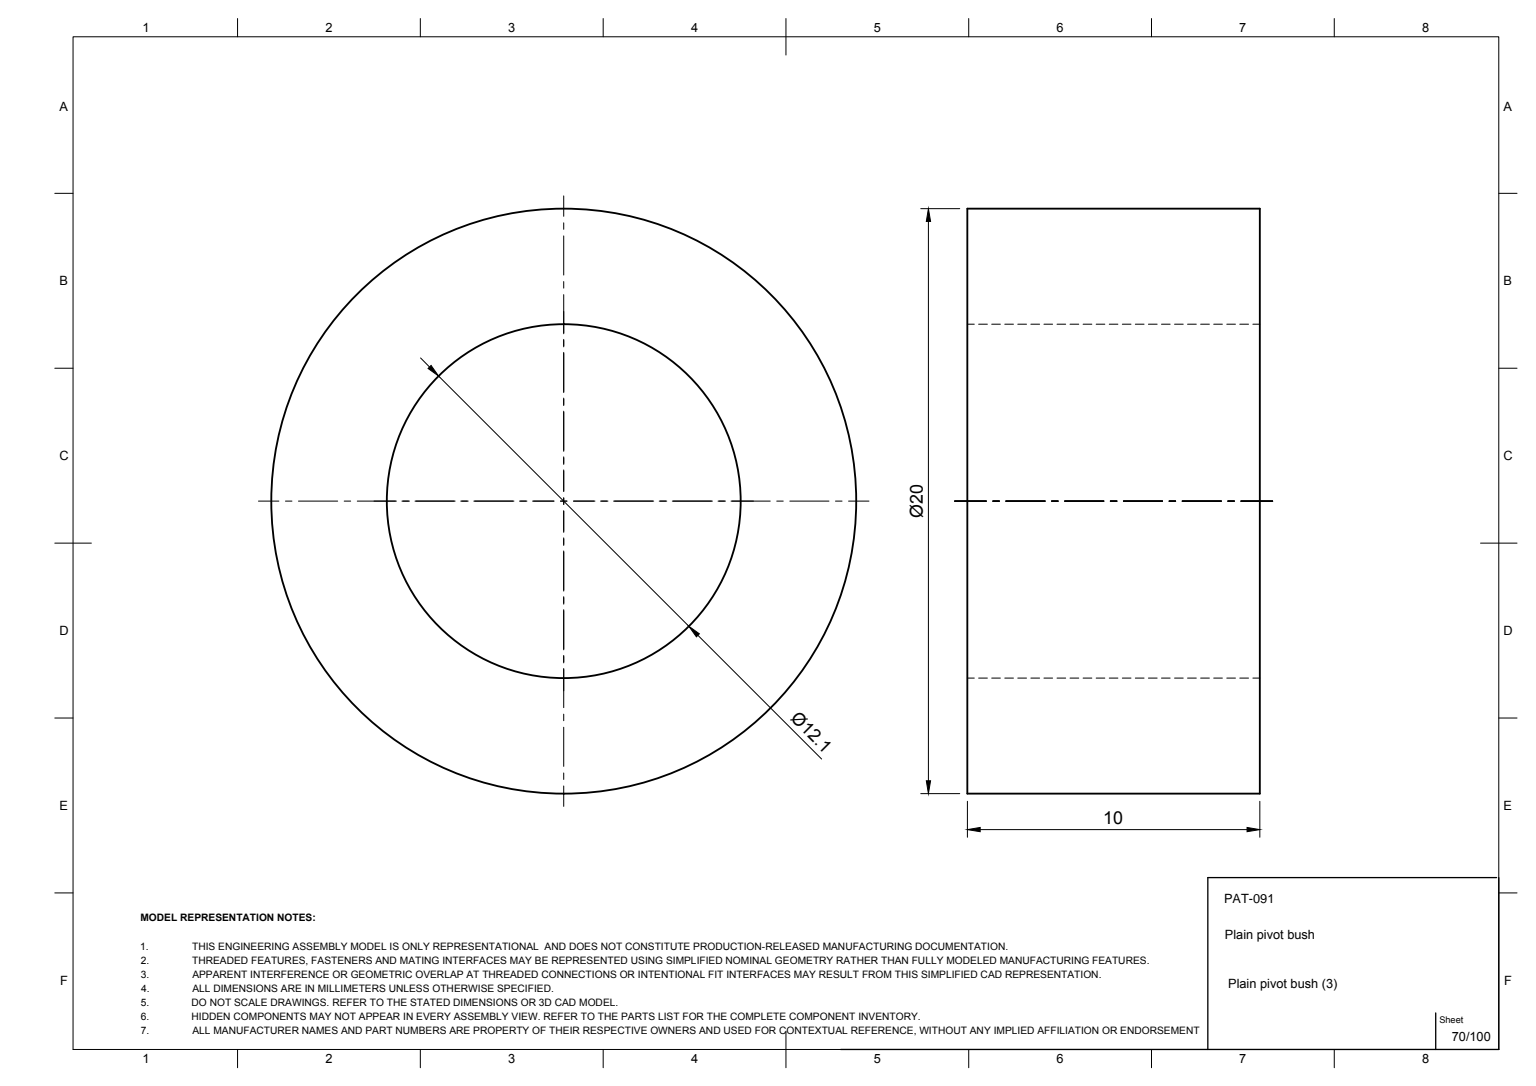
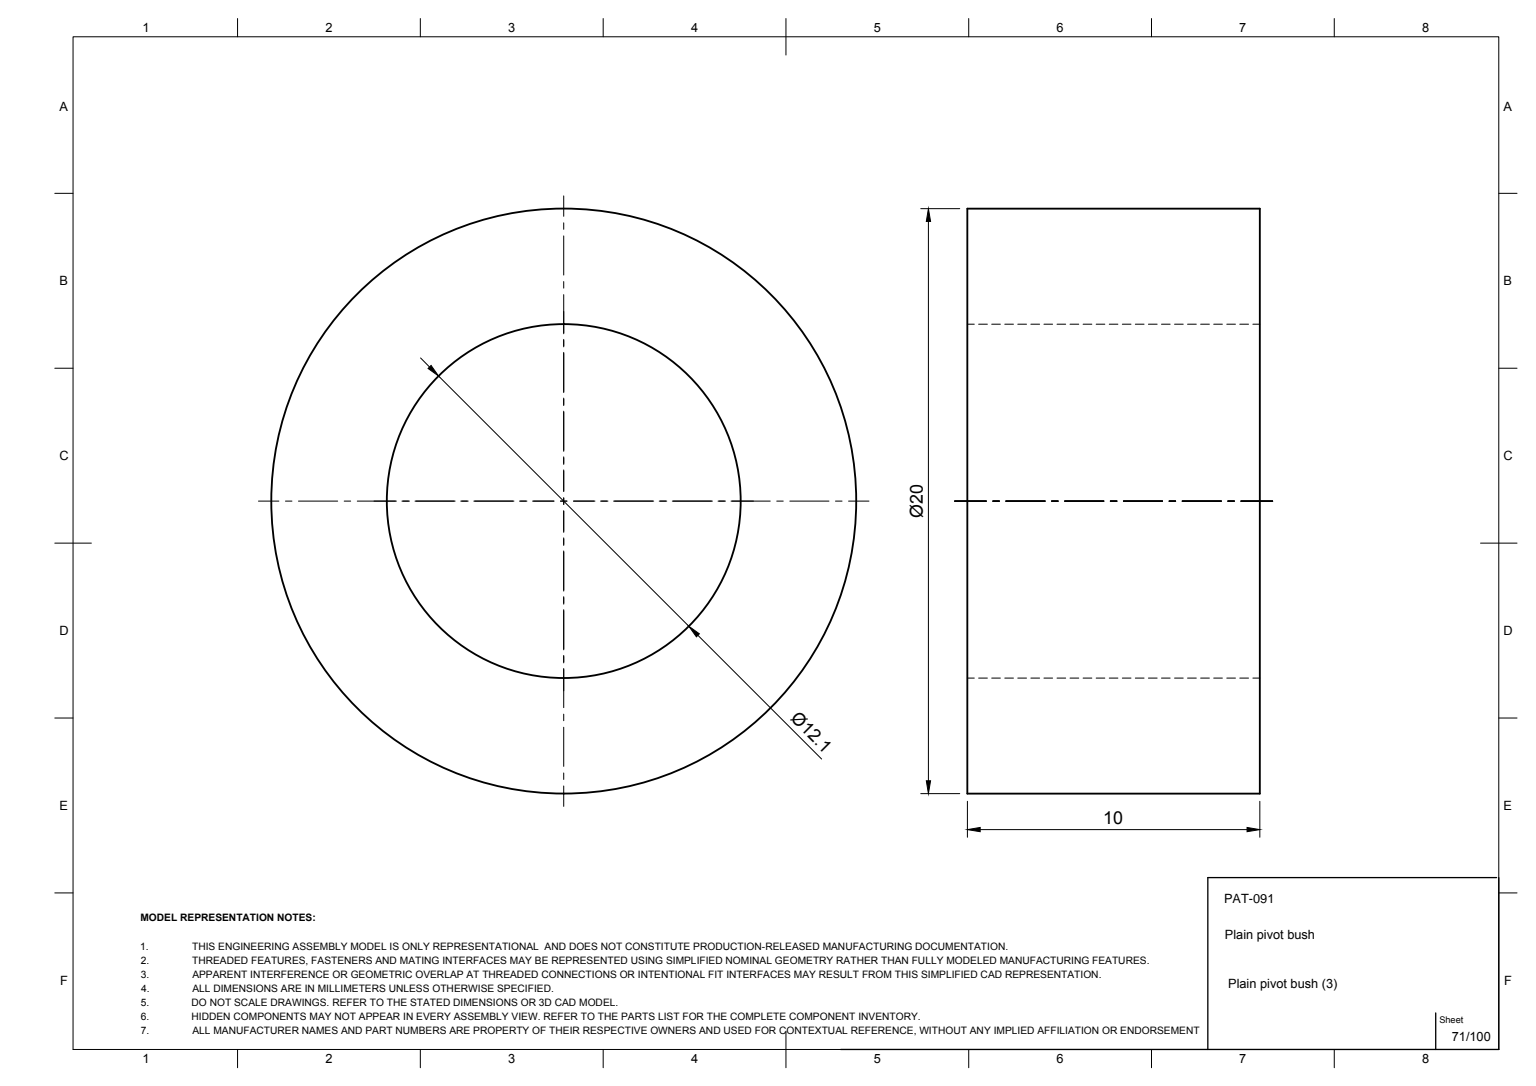
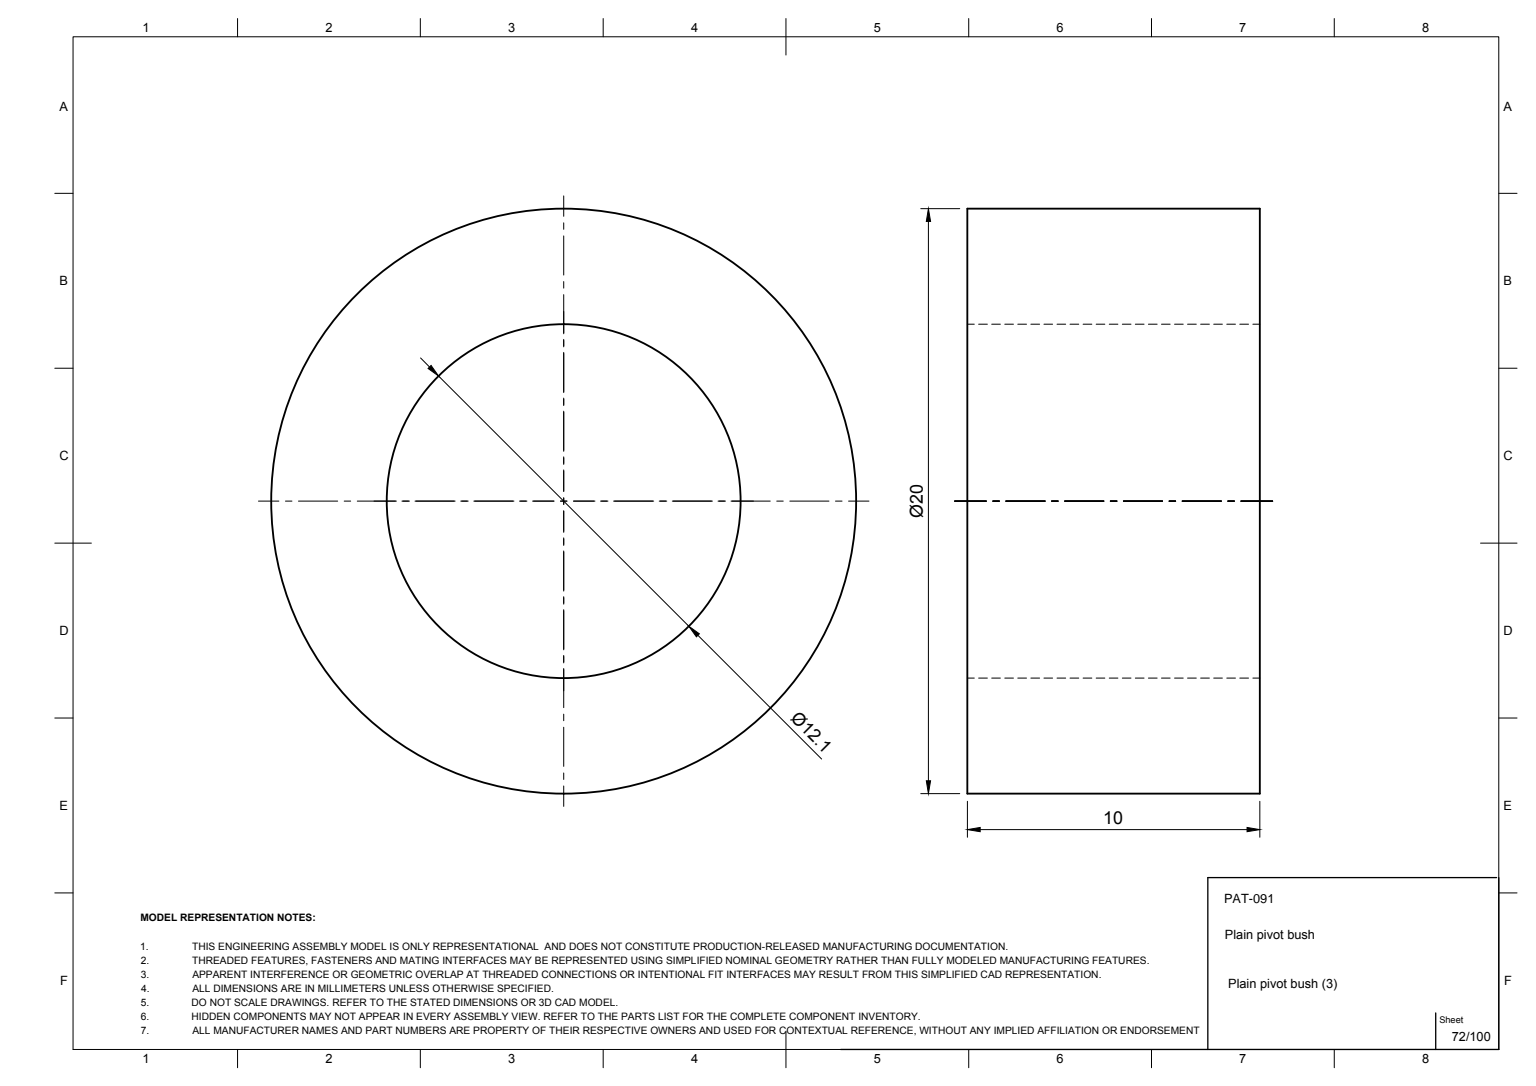
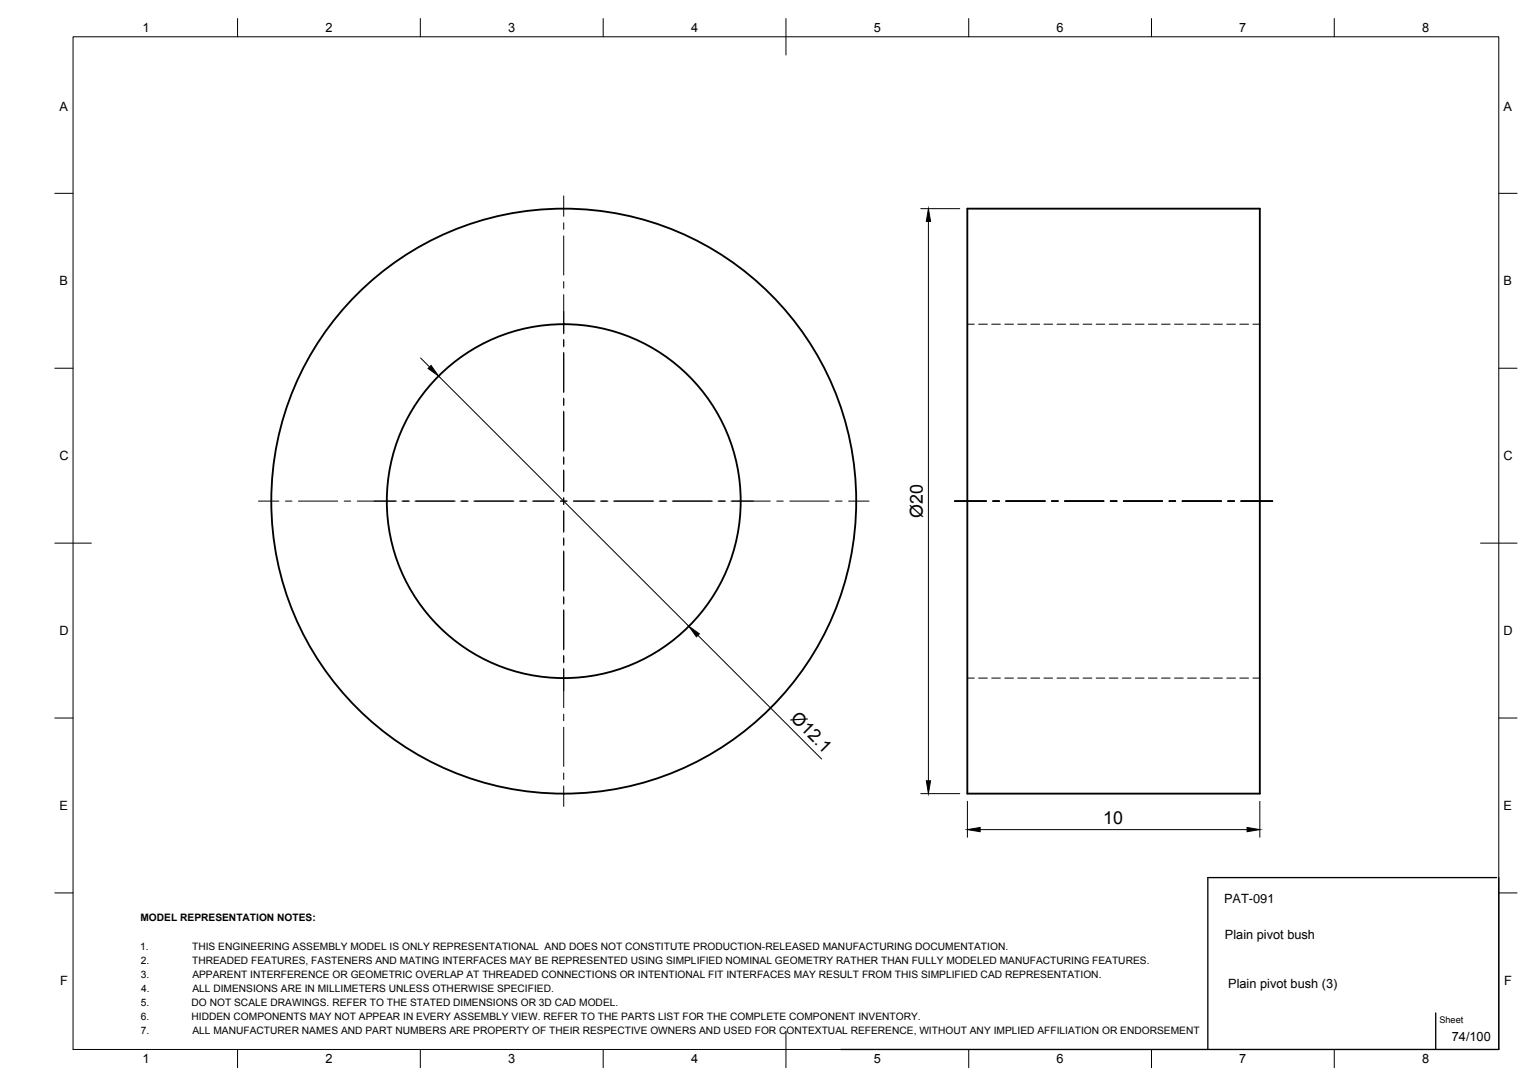
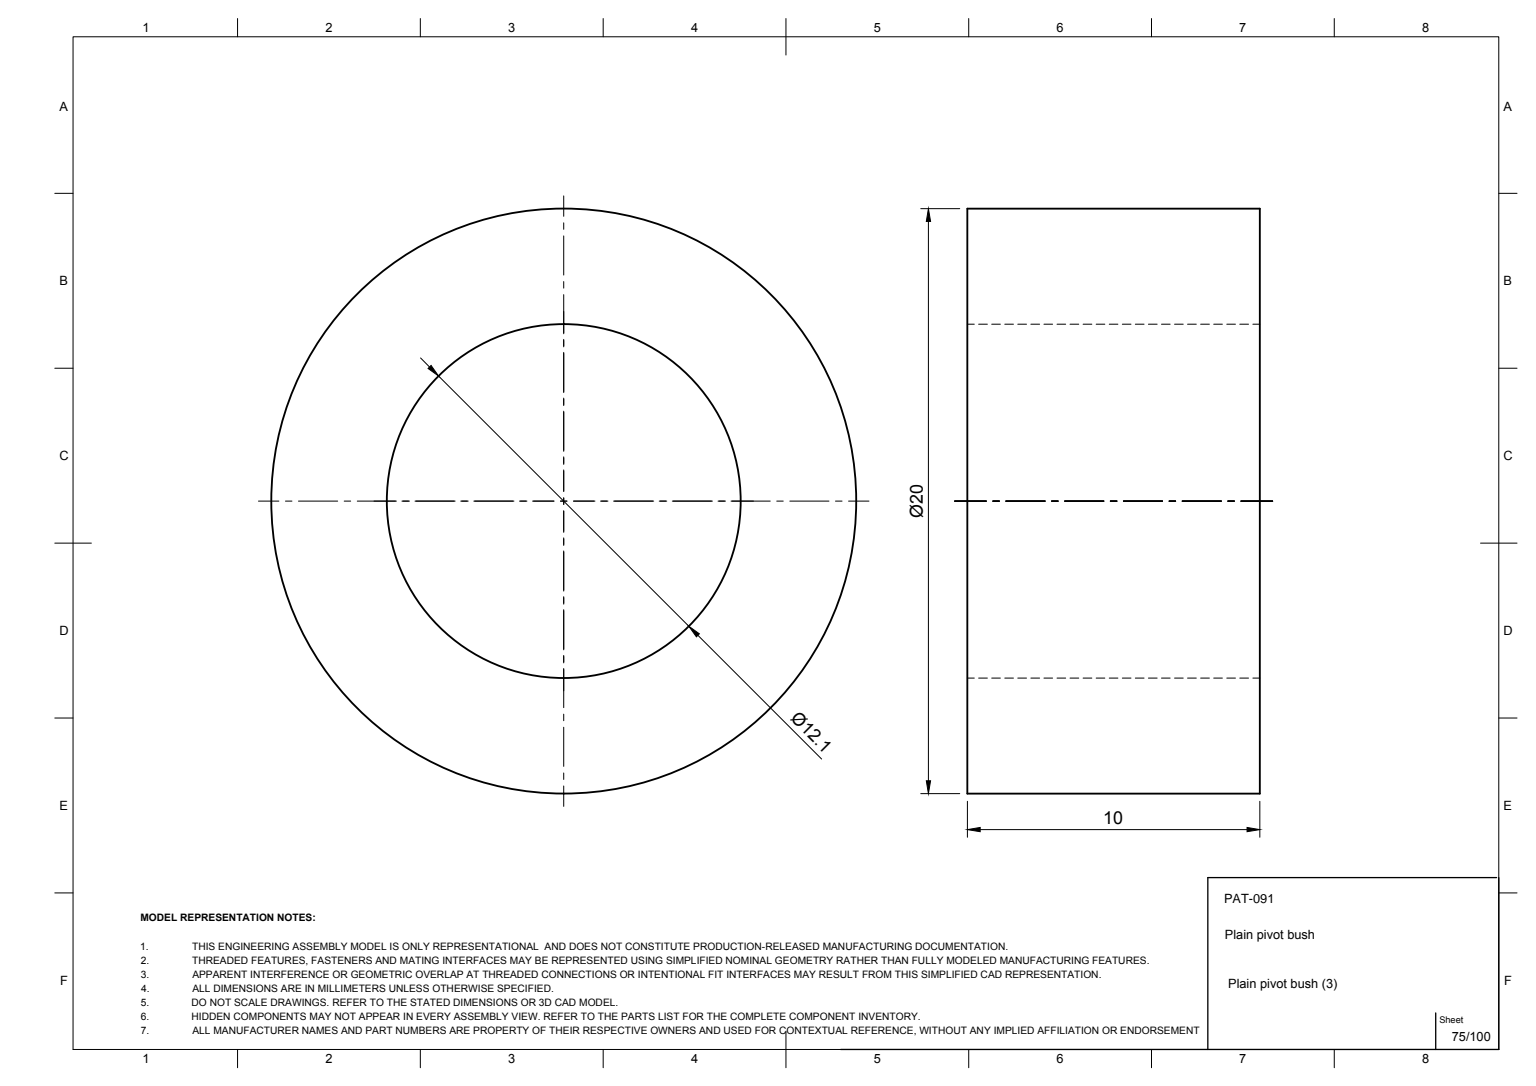
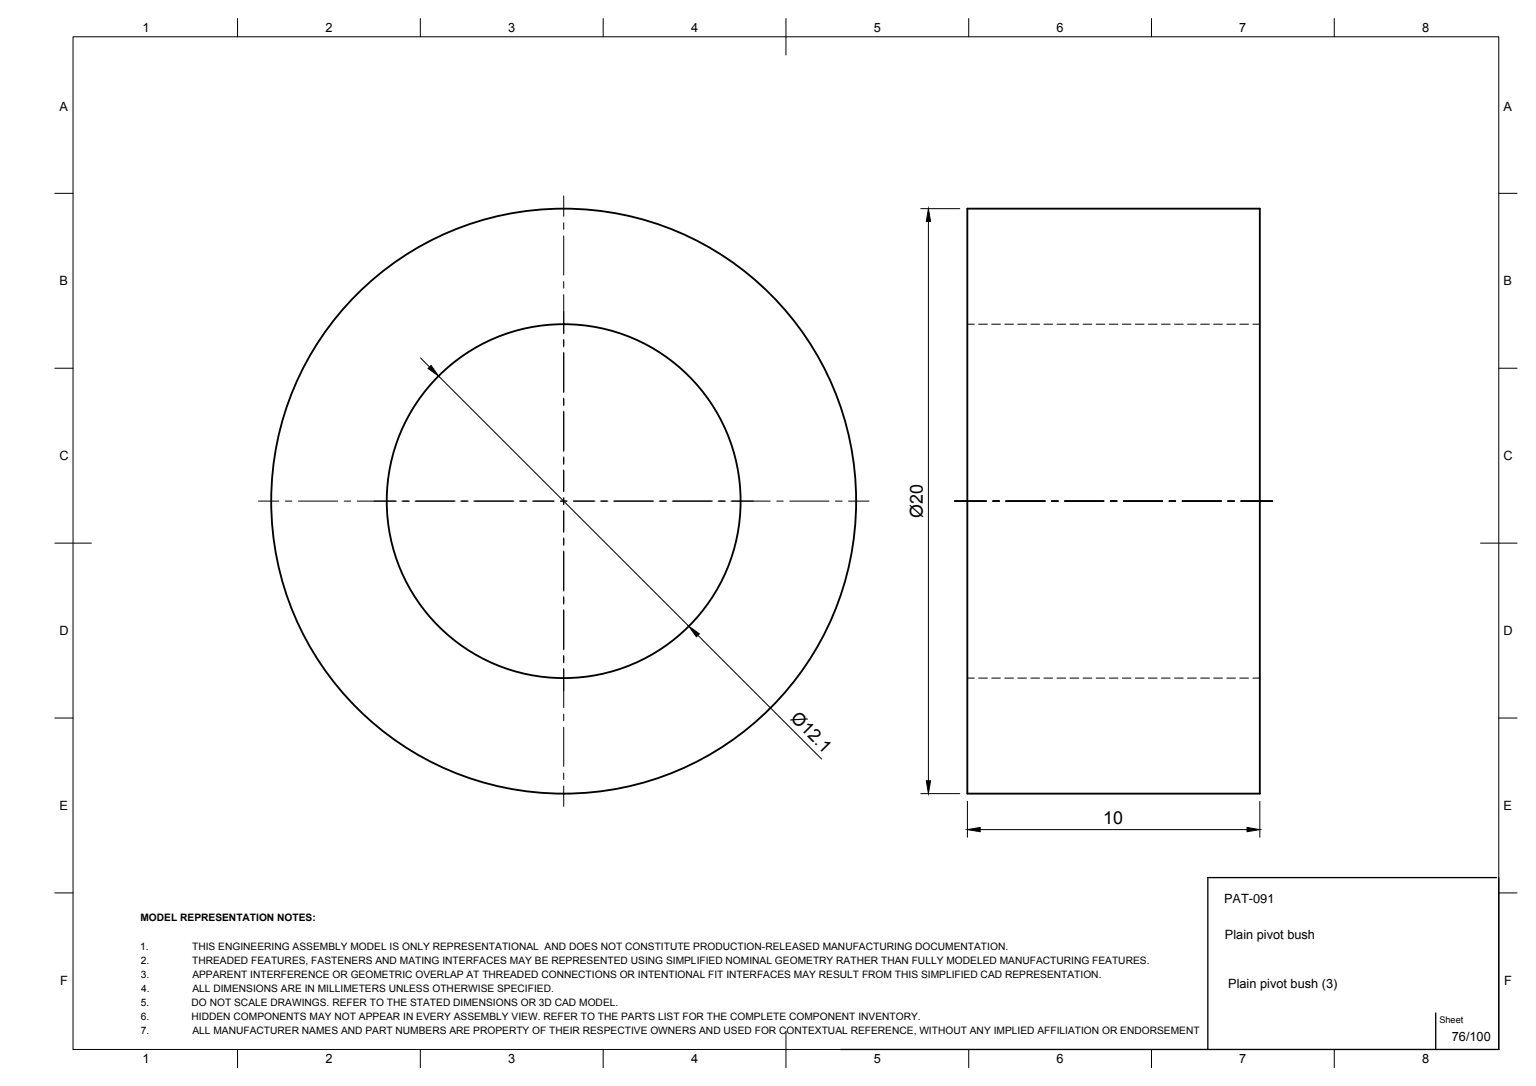
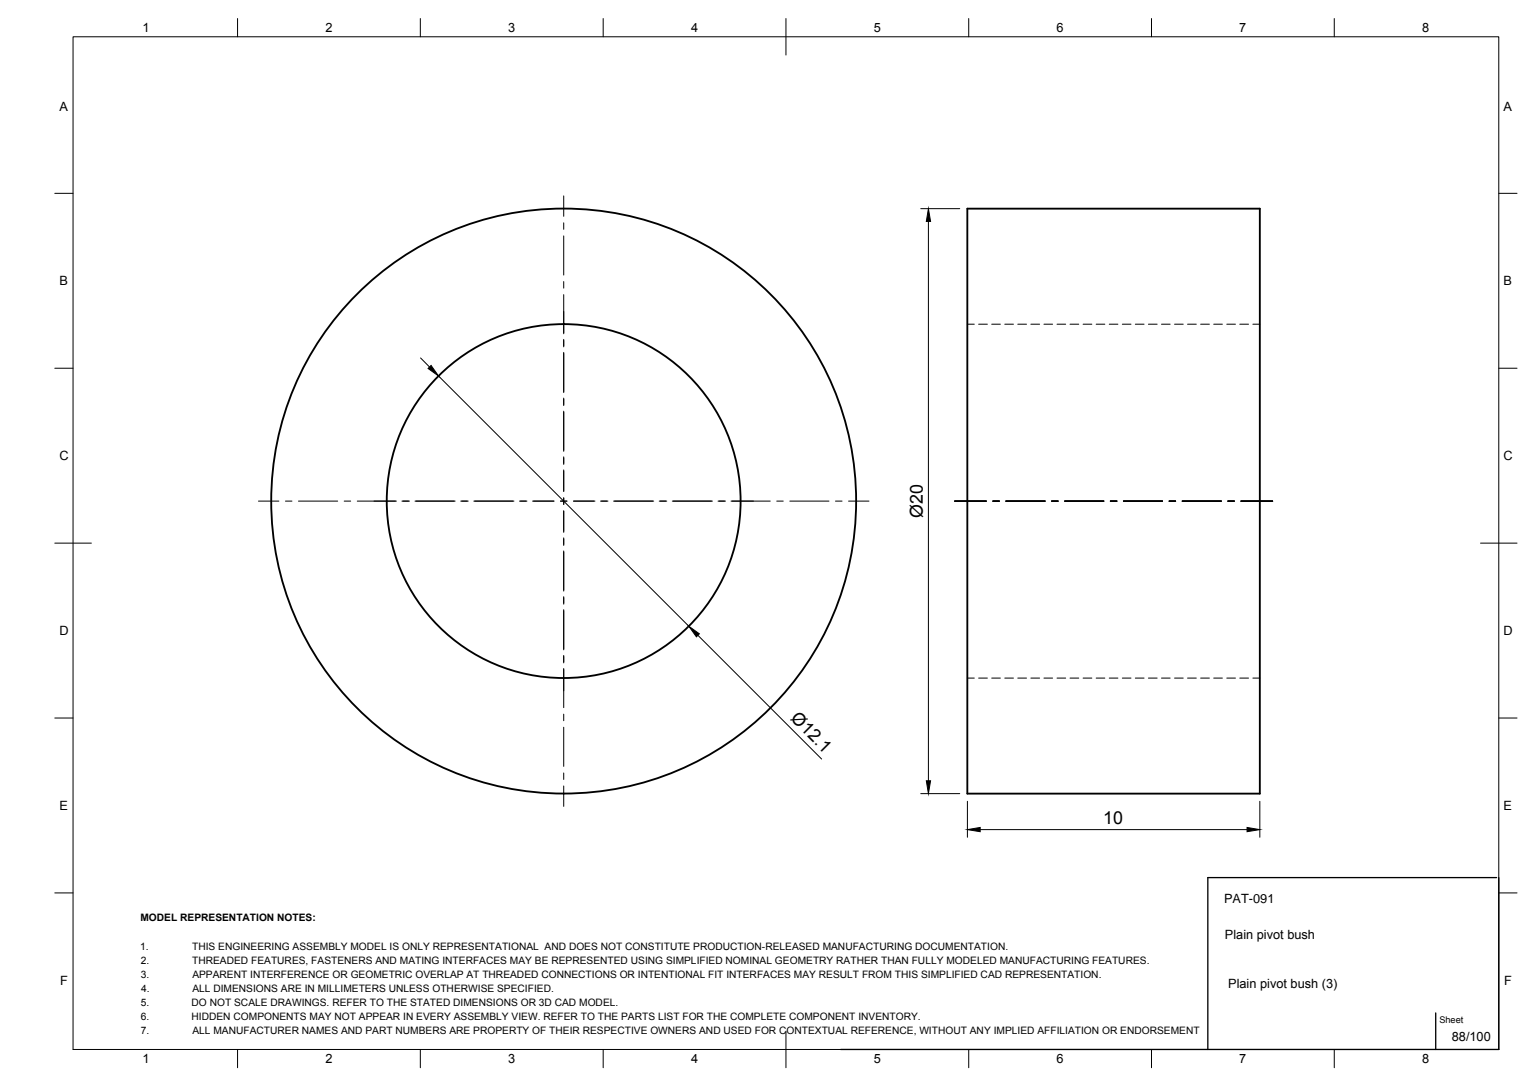
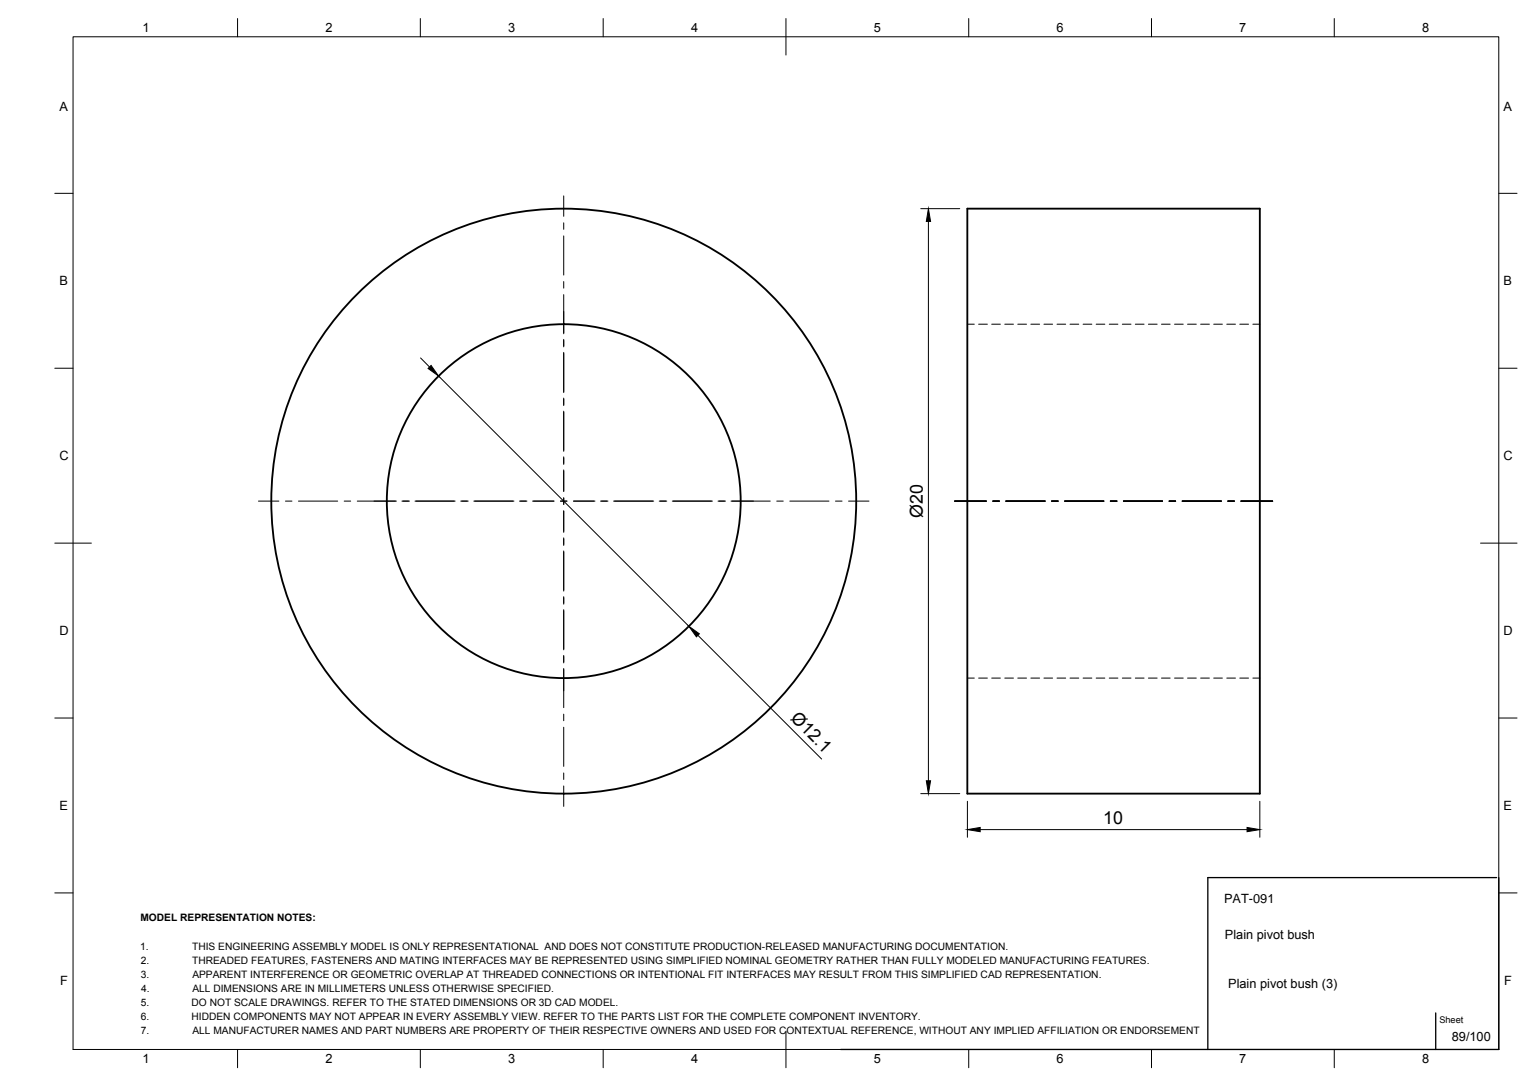
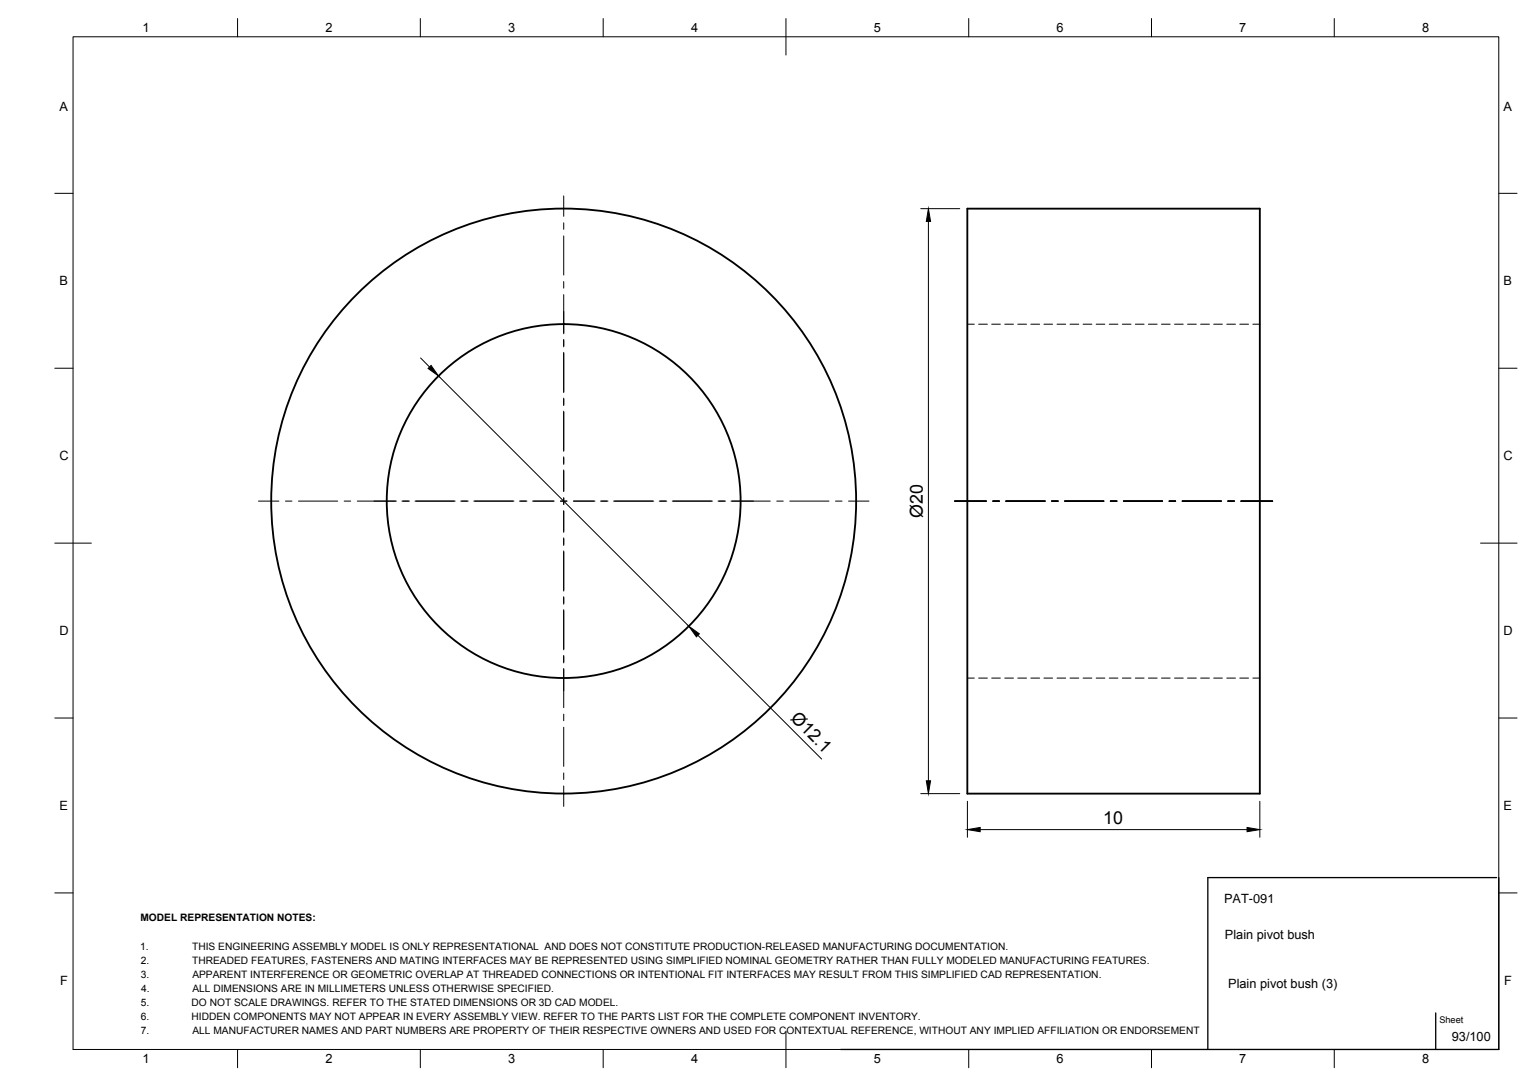
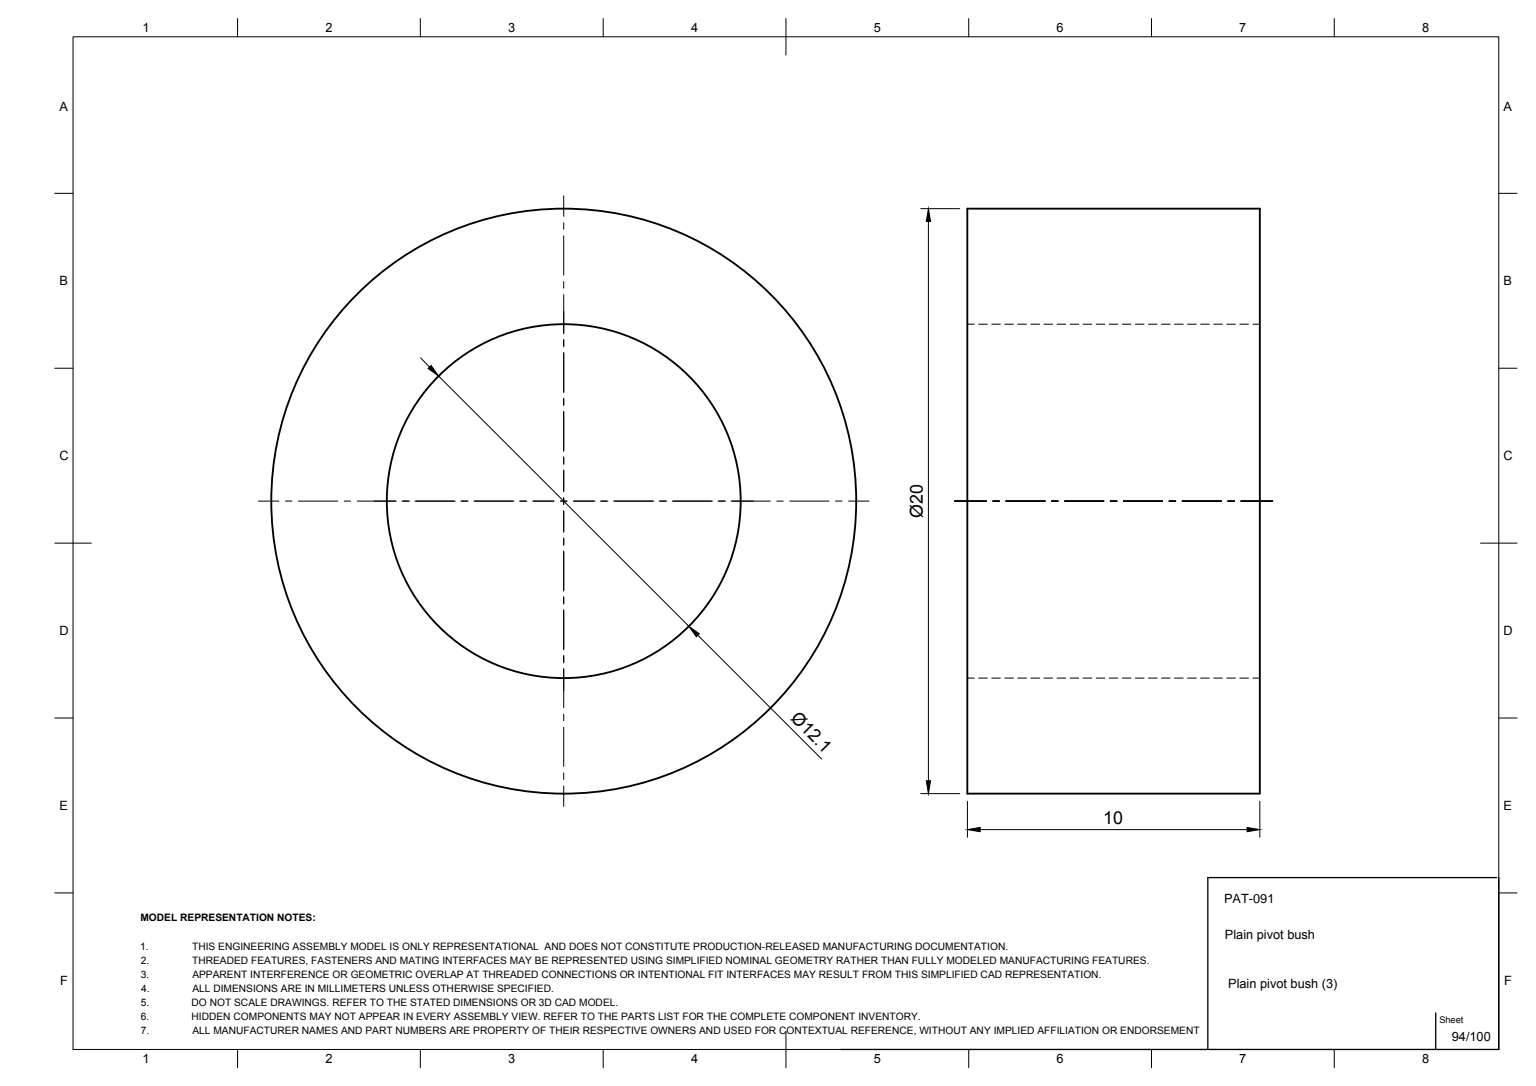
ISO-10303-21;
HEADER;
/* Generated by software containing ST-Developer
 * from STEP Tools, Inc. (www.steptools.com) 
 */

FILE_DESCRIPTION(
/* description */ ('PAT-091'),
/* implementation_level */ '2;1');

FILE_NAME(
/* name */ 'Plain pivot bush.step',
/* time_stamp */ '2026-10-27T15:34:44-07:00',
/* author */ (''),
/* organization */ (''),
/* preprocessor_version */ 'ST-DEVELOPER v20.2',
/* originating_system */ 'Autodesk Translation Framework v15.17.0.0',
/* authorisation */ '');

FILE_SCHEMA (('AUTOMOTIVE_DESIGN { 1 0 10303 214 3 1 1 }'));
ENDSEC;

DATA;
#10=MECHANICAL_DESIGN_GEOMETRIC_PRESENTATION_REPRESENTATION('',(#1028),#25100);
#808=SHAPE_REPRESENTATION_RELATIONSHIP('SRR','None',#25574,#918);
#918=ADVANCED_BREP_SHAPE_REPRESENTATION('',(#1150),#25044);
#1028=STYLED_ITEM('',(#26177),#1150);
#1150=MANIFOLD_SOLID_BREP('Body1',#13307);
#1490=FACE_BOUND('',#3620,.T.);
#1491=FACE_BOUND('',#3622,.T.);
#1901=PLANE('',#15521);
#1902=PLANE('',#15522);
#2524=FACE_OUTER_BOUND('',#3617,.T.);
#2525=FACE_OUTER_BOUND('',#3618,.T.);
#2526=FACE_OUTER_BOUND('',#3619,.T.);
#2527=FACE_OUTER_BOUND('',#3621,.T.);
#3617=EDGE_LOOP('',(#10840,#10841,#10842,#10843));
#3618=EDGE_LOOP('',(#10844,#10845,#10846,#10847));
#3619=EDGE_LOOP('',(#10848));
#3620=EDGE_LOOP('',(#10849));
#3621=EDGE_LOOP('',(#10850));
#3622=EDGE_LOOP('',(#10851));
#4652=LINE('',#23112,#5392);
#4653=LINE('',#23118,#5393);
#5392=VECTOR('',#18860,0.605);
#5393=VECTOR('',#18867,1.);
#6006=CIRCLE('',#15516,0.605);
#6007=CIRCLE('',#15517,0.605);
#6008=CIRCLE('',#15519,1.);
#6009=CIRCLE('',#15520,1.);
#7003=VERTEX_POINT('',#23109);
#7004=VERTEX_POINT('',#23111);
#7005=VERTEX_POINT('',#23115);
#7006=VERTEX_POINT('',#23117);
#8355=EDGE_CURVE('',#7003,#7003,#6006,.T.);
#8356=EDGE_CURVE('',#7003,#7004,#4652,.T.);
#8357=EDGE_CURVE('',#7004,#7004,#6007,.T.);
#8358=EDGE_CURVE('',#7005,#7005,#6008,.T.);
#8359=EDGE_CURVE('',#7005,#7006,#4653,.T.);
#8360=EDGE_CURVE('',#7006,#7006,#6009,.T.);
#10840=ORIENTED_EDGE('',*,*,#8355,.F.);
#10841=ORIENTED_EDGE('',*,*,#8356,.T.);
#10842=ORIENTED_EDGE('',*,*,#8357,.T.);
#10843=ORIENTED_EDGE('',*,*,#8356,.F.);
#10844=ORIENTED_EDGE('',*,*,#8358,.F.);
#10845=ORIENTED_EDGE('',*,*,#8359,.T.);
#10846=ORIENTED_EDGE('',*,*,#8360,.T.);
#10847=ORIENTED_EDGE('',*,*,#8359,.F.);
#10848=ORIENTED_EDGE('',*,*,#8358,.T.);
#10849=ORIENTED_EDGE('',*,*,#8355,.T.);
#10850=ORIENTED_EDGE('',*,*,#8360,.F.);
#10851=ORIENTED_EDGE('',*,*,#8357,.F.);
#12266=CYLINDRICAL_SURFACE('',#15515,0.605);
#12267=CYLINDRICAL_SURFACE('',#15518,1.);
#12891=ADVANCED_FACE('',(#2524),#12266,.F.);
#12892=ADVANCED_FACE('',(#2525),#12267,.T.);
#12893=ADVANCED_FACE('',(#2526,#1490),#1901,.T.);
#12894=ADVANCED_FACE('',(#2527,#1491),#1902,.F.);
#13307=CLOSED_SHELL('',(#12891,#12892,#12893,#12894));
#15514=AXIS2_PLACEMENT_3D('',#23107,#18854,#18855);
#15515=AXIS2_PLACEMENT_3D('',#23108,#18856,#18857);
#15516=AXIS2_PLACEMENT_3D('',#23110,#18858,#18859);
#15517=AXIS2_PLACEMENT_3D('',#23113,#18861,#18862);
#15518=AXIS2_PLACEMENT_3D('',#23114,#18863,#18864);
#15519=AXIS2_PLACEMENT_3D('',#23116,#18865,#18866);
#15520=AXIS2_PLACEMENT_3D('',#23119,#18868,#18869);
#15521=AXIS2_PLACEMENT_3D('',#23120,#18870,#18871);
#15522=AXIS2_PLACEMENT_3D('',#23121,#18872,#18873);
#18854=DIRECTION('axis',(0.,0.,1.));
#18855=DIRECTION('refdir',(1.,0.,0.));
#18856=DIRECTION('center_axis',(0.,1.,0.));
#18857=DIRECTION('ref_axis',(1.,0.,0.));
#18858=DIRECTION('center_axis',(0.,-1.,0.));
#18859=DIRECTION('ref_axis',(1.,0.,0.));
#18860=DIRECTION('',(0.,-1.,0.));
#18861=DIRECTION('center_axis',(0.,-1.,0.));
#18862=DIRECTION('ref_axis',(1.,0.,0.));
#18863=DIRECTION('center_axis',(0.,1.,0.));
#18864=DIRECTION('ref_axis',(1.,0.,0.));
#18865=DIRECTION('center_axis',(0.,1.,0.));
#18866=DIRECTION('ref_axis',(1.,0.,0.));
#18867=DIRECTION('',(0.,-1.,0.));
#18868=DIRECTION('center_axis',(0.,1.,0.));
#18869=DIRECTION('ref_axis',(1.,0.,0.));
#18870=DIRECTION('center_axis',(0.,1.,0.));
#18871=DIRECTION('ref_axis',(1.,0.,0.));
#18872=DIRECTION('center_axis',(0.,1.,0.));
#18873=DIRECTION('ref_axis',(1.,0.,0.));
#23107=CARTESIAN_POINT('',(0.,0.,0.));
#23108=CARTESIAN_POINT('Origin',(0.,-7.,3.));
#23109=CARTESIAN_POINT('',(-0.605,-6.,3.));
#23110=CARTESIAN_POINT('Origin',(0.,-6.,3.));
#23111=CARTESIAN_POINT('',(-0.605,-7.,3.));
#23112=CARTESIAN_POINT('',(-0.605,-7.,3.));
#23113=CARTESIAN_POINT('Origin',(0.,-7.,3.));
#23114=CARTESIAN_POINT('Origin',(0.,-7.,3.));
#23115=CARTESIAN_POINT('',(-1.,-6.,3.));
#23116=CARTESIAN_POINT('Origin',(0.,-6.,3.));
#23117=CARTESIAN_POINT('',(-1.,-7.,3.));
#23118=CARTESIAN_POINT('',(-1.,-7.,3.));
#23119=CARTESIAN_POINT('Origin',(0.,-7.,3.));
#23120=CARTESIAN_POINT('Origin',(0.,-6.,3.));
#23121=CARTESIAN_POINT('Origin',(0.,-7.,3.));
#24923=UNCERTAINTY_MEASURE_WITH_UNIT(LENGTH_MEASURE(0.001),#25101,
'DISTANCE_ACCURACY_VALUE',
'Maximum model space distance between geometric entities at asserted c
onnectivities');
#24979=UNCERTAINTY_MEASURE_WITH_UNIT(LENGTH_MEASURE(0.001),#25101,
'DISTANCE_ACCURACY_VALUE',
'Maximum model space distance between geometric entities at asserted c
onnectivities');
#25044=(
GEOMETRIC_REPRESENTATION_CONTEXT(3)
GLOBAL_UNCERTAINTY_ASSIGNED_CONTEXT((#24923))
GLOBAL_UNIT_ASSIGNED_CONTEXT((#25101,#25103,#25104))
REPRESENTATION_CONTEXT('','3D')
);
#25100=(
GEOMETRIC_REPRESENTATION_CONTEXT(3)
GLOBAL_UNCERTAINTY_ASSIGNED_CONTEXT((#24979))
GLOBAL_UNIT_ASSIGNED_CONTEXT((#25101,#25103,#25104))
REPRESENTATION_CONTEXT('','3D')
);
#25101=(
LENGTH_UNIT()
NAMED_UNIT(*)
SI_UNIT(.CENTI.,.METRE.)
);
#25103=(
NAMED_UNIT(*)
PLANE_ANGLE_UNIT()
SI_UNIT($,.RADIAN.)
);
#25104=(
NAMED_UNIT(*)
SI_UNIT($,.STERADIAN.)
SOLID_ANGLE_UNIT()
);
#25169=SHAPE_DEFINITION_REPRESENTATION(#25291,#25574);
#25291=PRODUCT_DEFINITION_SHAPE('',$,#25695);
#25574=SHAPE_REPRESENTATION('',(#15514),#25044);
#25630=PRODUCT_DEFINITION_CONTEXT('part definition',#25992,'design');
#25695=PRODUCT_DEFINITION('Plain pivot bush','Plain pivot bush',#25815,
#25630);
#25815=PRODUCT_DEFINITION_FORMATION('',$,#26058);
#25992=APPLICATION_CONTEXT(
'Core Data for Automotive Mechanical Design Process');
#25993=PRODUCT_CONTEXT('part definition',#25992,'mechanical');
#26058=PRODUCT('Plain pivot bush','Plain pivot bush','Plain pivot bush',
(#25993));
#26171=COLOUR_RGB('Light Blue',0.38,0.62,0.78);
#26172=FILL_AREA_STYLE_COLOUR('',#26171);
#26173=FILL_AREA_STYLE('',(#26172));
#26174=SURFACE_STYLE_FILL_AREA(#26173);
#26175=SURFACE_SIDE_STYLE('',(#26174));
#26176=SURFACE_STYLE_USAGE(.BOTH.,#26175);
#26177=PRESENTATION_STYLE_ASSIGNMENT((#26176));
ENDSEC;
END-ISO-10303-21;
